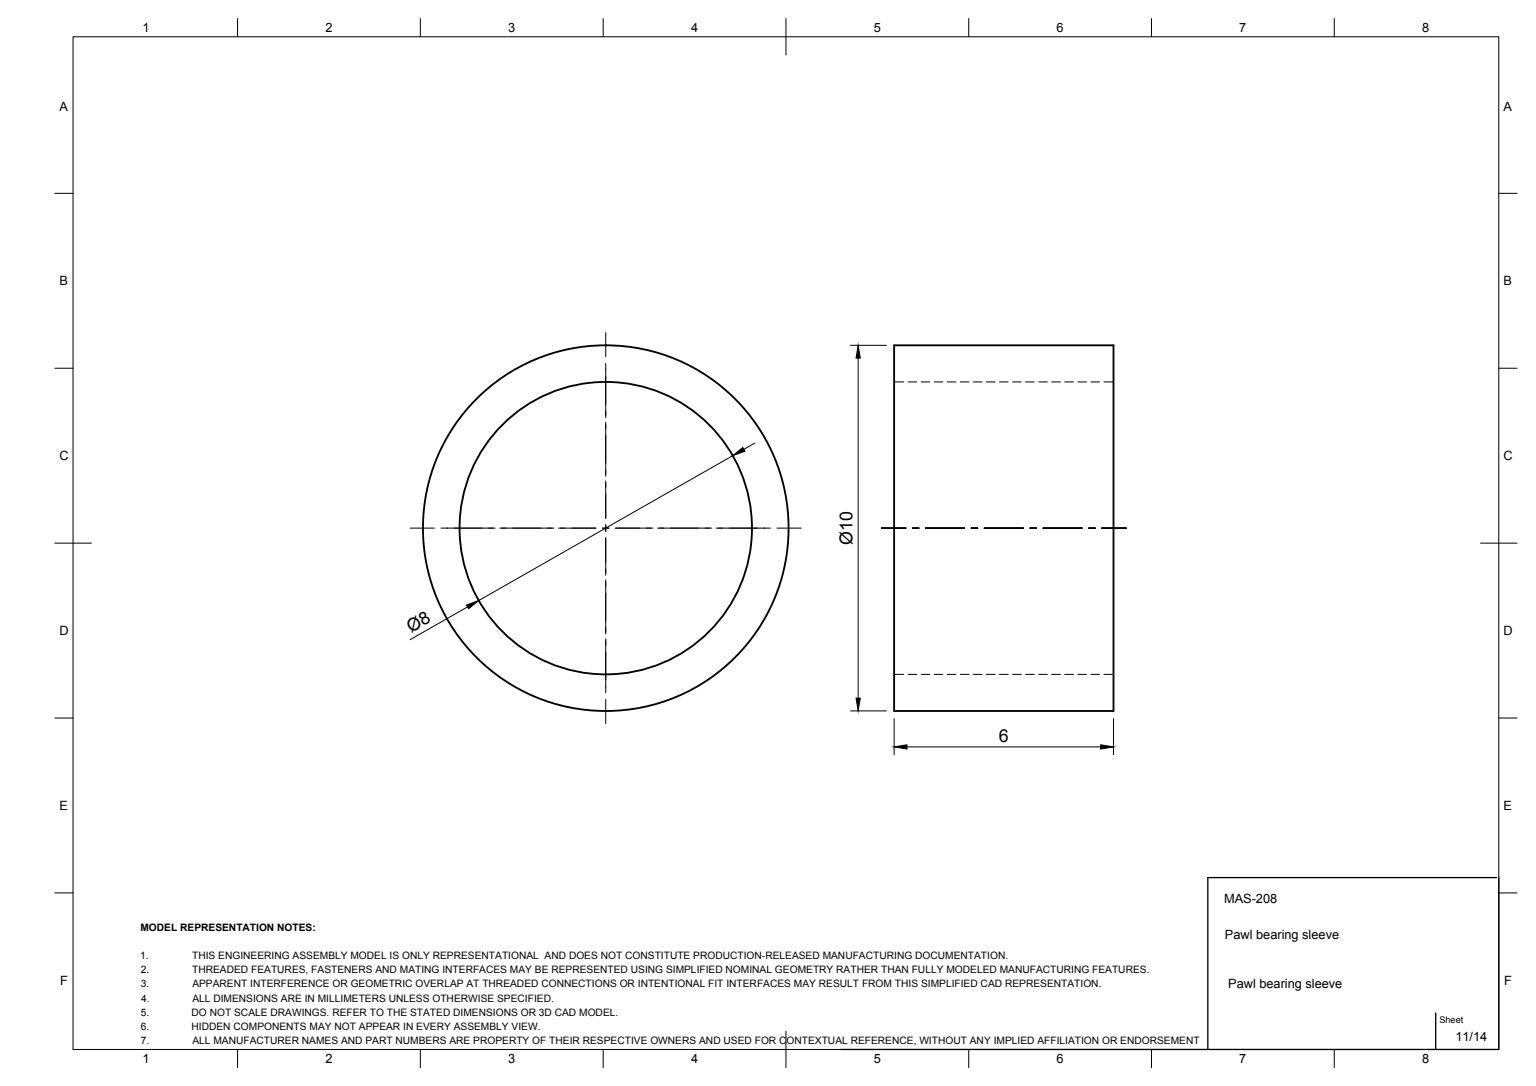
ISO-10303-21;
HEADER;
/* Generated by software containing ST-Developer
 * from STEP Tools, Inc. (www.steptools.com) 
 */

FILE_DESCRIPTION(
/* description */ ('Independent vertical20-tooth ratchet advance with repeated integral-c
ounterweight gravity pawls, swinging drive lever, bronze sleeves and f
ully retained axle stacks.18degpertooth. Native revolutes; geometric c
ycle checking rather than automatic contact/rolling dynamics. Gravity 
closing checked from actual pawl center of mass. Backplate/foot suppor
ts unit. Fits, torque, holding force, wear and life unassigned.'),
/* implementation_level */ '2;1');

FILE_NAME(
/* name */ 'Pawl bearing sleeve.step',
/* time_stamp */ '2026-11-09T06:25:53-08:00',
/* author */ (''),
/* organization */ (''),
/* preprocessor_version */ 'ST-DEVELOPER v20.2',
/* originating_system */ 'Autodesk Translation Framework v15.17.0.0',
/* authorisation */ '');

FILE_SCHEMA (('AUTOMOTIVE_DESIGN { 1 0 10303 214 3 1 1 }'));
ENDSEC;

DATA;
#10=MECHANICAL_DESIGN_GEOMETRIC_PRESENTATION_REPRESENTATION('',(#132),#4643);
#104=SHAPE_REPRESENTATION_RELATIONSHIP('SRR','None',#4709,#118);
#118=ADVANCED_BREP_SHAPE_REPRESENTATION('',(#146),#4638);
#132=STYLED_ITEM('',(#4785),#146);
#146=MANIFOLD_SOLID_BREP('Body1',#2668);
#184=FACE_BOUND('',#616,.T.);
#185=FACE_BOUND('',#618,.T.);
#292=PLANE('',#3026);
#293=PLANE('',#3027);
#431=FACE_OUTER_BOUND('',#613,.T.);
#432=FACE_OUTER_BOUND('',#614,.T.);
#433=FACE_OUTER_BOUND('',#615,.T.);
#434=FACE_OUTER_BOUND('',#617,.T.);
#613=EDGE_LOOP('',(#2401,#2402,#2403,#2404));
#614=EDGE_LOOP('',(#2405,#2406,#2407,#2408));
#615=EDGE_LOOP('',(#2409));
#616=EDGE_LOOP('',(#2410));
#617=EDGE_LOOP('',(#2411));
#618=EDGE_LOOP('',(#2412));
#889=LINE('',#4509,#1151);
#890=LINE('',#4515,#1152);
#1151=VECTOR('',#3721,4.);
#1152=VECTOR('',#3728,5.);
#1221=CIRCLE('',#3021,4.);
#1222=CIRCLE('',#3022,4.);
#1223=CIRCLE('',#3024,5.);
#1224=CIRCLE('',#3025,5.);
#1441=VERTEX_POINT('',#4506);
#1442=VERTEX_POINT('',#4508);
#1443=VERTEX_POINT('',#4512);
#1444=VERTEX_POINT('',#4514);
#1765=EDGE_CURVE('',#1441,#1441,#1221,.T.);
#1766=EDGE_CURVE('',#1441,#1442,#889,.T.);
#1767=EDGE_CURVE('',#1442,#1442,#1222,.T.);
#1768=EDGE_CURVE('',#1443,#1443,#1223,.T.);
#1769=EDGE_CURVE('',#1443,#1444,#890,.T.);
#1770=EDGE_CURVE('',#1444,#1444,#1224,.T.);
#2401=ORIENTED_EDGE('',*,*,#1765,.F.);
#2402=ORIENTED_EDGE('',*,*,#1766,.T.);
#2403=ORIENTED_EDGE('',*,*,#1767,.T.);
#2404=ORIENTED_EDGE('',*,*,#1766,.F.);
#2405=ORIENTED_EDGE('',*,*,#1768,.F.);
#2406=ORIENTED_EDGE('',*,*,#1769,.T.);
#2407=ORIENTED_EDGE('',*,*,#1770,.T.);
#2408=ORIENTED_EDGE('',*,*,#1769,.F.);
#2409=ORIENTED_EDGE('',*,*,#1768,.T.);
#2410=ORIENTED_EDGE('',*,*,#1765,.T.);
#2411=ORIENTED_EDGE('',*,*,#1770,.F.);
#2412=ORIENTED_EDGE('',*,*,#1767,.F.);
#2500=CYLINDRICAL_SURFACE('',#3020,4.);
#2501=CYLINDRICAL_SURFACE('',#3023,5.);
#2637=ADVANCED_FACE('',(#431),#2500,.F.);
#2638=ADVANCED_FACE('',(#432),#2501,.T.);
#2639=ADVANCED_FACE('',(#433,#184),#292,.T.);
#2640=ADVANCED_FACE('',(#434,#185),#293,.F.);
#2668=CLOSED_SHELL('',(#2637,#2638,#2639,#2640));
#3019=AXIS2_PLACEMENT_3D('',#4504,#3715,#3716);
#3020=AXIS2_PLACEMENT_3D('',#4505,#3717,#3718);
#3021=AXIS2_PLACEMENT_3D('',#4507,#3719,#3720);
#3022=AXIS2_PLACEMENT_3D('',#4510,#3722,#3723);
#3023=AXIS2_PLACEMENT_3D('',#4511,#3724,#3725);
#3024=AXIS2_PLACEMENT_3D('',#4513,#3726,#3727);
#3025=AXIS2_PLACEMENT_3D('',#4516,#3729,#3730);
#3026=AXIS2_PLACEMENT_3D('',#4517,#3731,#3732);
#3027=AXIS2_PLACEMENT_3D('',#4518,#3733,#3734);
#3715=DIRECTION('axis',(0.,0.,1.));
#3716=DIRECTION('refdir',(1.,0.,0.));
#3717=DIRECTION('center_axis',(0.,0.,1.));
#3718=DIRECTION('ref_axis',(1.,0.,0.));
#3719=DIRECTION('center_axis',(0.,0.,-1.));
#3720=DIRECTION('ref_axis',(1.,0.,0.));
#3721=DIRECTION('',(0.,0.,-1.));
#3722=DIRECTION('center_axis',(0.,0.,-1.));
#3723=DIRECTION('ref_axis',(1.,0.,0.));
#3724=DIRECTION('center_axis',(0.,0.,1.));
#3725=DIRECTION('ref_axis',(1.,0.,0.));
#3726=DIRECTION('center_axis',(0.,0.,1.));
#3727=DIRECTION('ref_axis',(1.,0.,0.));
#3728=DIRECTION('',(0.,0.,-1.));
#3729=DIRECTION('center_axis',(0.,0.,1.));
#3730=DIRECTION('ref_axis',(1.,0.,0.));
#3731=DIRECTION('center_axis',(0.,0.,1.));
#3732=DIRECTION('ref_axis',(1.,0.,0.));
#3733=DIRECTION('center_axis',(0.,0.,1.));
#3734=DIRECTION('ref_axis',(1.,0.,0.));
#4504=CARTESIAN_POINT('',(0.,0.,0.));
#4505=CARTESIAN_POINT('Origin',(0.,0.,0.));
#4506=CARTESIAN_POINT('',(-4.,-4.89858719658941E-16,6.));
#4507=CARTESIAN_POINT('Origin',(0.,0.,6.));
#4508=CARTESIAN_POINT('',(-4.,-4.89858719658941E-16,0.));
#4509=CARTESIAN_POINT('',(-4.,-4.89858719658941E-16,0.));
#4510=CARTESIAN_POINT('Origin',(0.,0.,0.));
#4511=CARTESIAN_POINT('Origin',(0.,0.,0.));
#4512=CARTESIAN_POINT('',(-5.,-6.12323399573677E-16,6.));
#4513=CARTESIAN_POINT('Origin',(0.,0.,6.));
#4514=CARTESIAN_POINT('',(-5.,-6.12323399573677E-16,0.));
#4515=CARTESIAN_POINT('',(-5.,-6.12323399573677E-16,0.));
#4516=CARTESIAN_POINT('Origin',(0.,0.,0.));
#4517=CARTESIAN_POINT('Origin',(0.,0.,6.));
#4518=CARTESIAN_POINT('Origin',(0.,0.,0.));
#4622=UNCERTAINTY_MEASURE_WITH_UNIT(LENGTH_MEASURE(0.01),#4644,
'DISTANCE_ACCURACY_VALUE',
'Maximum model space distance between geometric entities at asserted c
onnectivities');
#4627=UNCERTAINTY_MEASURE_WITH_UNIT(LENGTH_MEASURE(0.01),#4644,
'DISTANCE_ACCURACY_VALUE',
'Maximum model space distance between geometric entities at asserted c
onnectivities');
#4638=(
GEOMETRIC_REPRESENTATION_CONTEXT(3)
GLOBAL_UNCERTAINTY_ASSIGNED_CONTEXT((#4622))
GLOBAL_UNIT_ASSIGNED_CONTEXT((#4644,#4646,#4647))
REPRESENTATION_CONTEXT('','3D')
);
#4643=(
GEOMETRIC_REPRESENTATION_CONTEXT(3)
GLOBAL_UNCERTAINTY_ASSIGNED_CONTEXT((#4627))
GLOBAL_UNIT_ASSIGNED_CONTEXT((#4644,#4646,#4647))
REPRESENTATION_CONTEXT('','3D')
);
#4644=(
LENGTH_UNIT()
NAMED_UNIT(*)
SI_UNIT(.MILLI.,.METRE.)
);
#4646=(
NAMED_UNIT(*)
PLANE_ANGLE_UNIT()
SI_UNIT($,.RADIAN.)
);
#4647=(
NAMED_UNIT(*)
SI_UNIT($,.STERADIAN.)
SOLID_ANGLE_UNIT()
);
#4658=SHAPE_DEFINITION_REPRESENTATION(#4673,#4709);
#4673=PRODUCT_DEFINITION_SHAPE('',$,#4725);
#4709=SHAPE_REPRESENTATION('',(#3019),#4638);
#4714=PRODUCT_DEFINITION_CONTEXT('part definition',#4761,'design');
#4725=PRODUCT_DEFINITION('Pawl bearing sleeve','Pawl bearing sleeve',#4740,
#4714);
#4740=PRODUCT_DEFINITION_FORMATION('',$,#4773);
#4761=APPLICATION_CONTEXT(
'Core Data for Automotive Mechanical Design Process');
#4762=PRODUCT_CONTEXT('part definition',#4761,'mechanical');
#4773=PRODUCT('Pawl bearing sleeve','Pawl bearing sleeve',$,(#4762));
#4785=PRESENTATION_STYLE_ASSIGNMENT((#4794));
#4794=SURFACE_STYLE_USAGE(.BOTH.,#4803);
#4803=SURFACE_SIDE_STYLE('',(#4812));
#4812=SURFACE_STYLE_FILL_AREA(#4821);
#4821=FILL_AREA_STYLE('Bearing light gray',(#4830));
#4830=FILL_AREA_STYLE_COLOUR('Bearing light gray',#4839);
#4839=COLOUR_RGB('Bearing light gray',0.725490196078431,0.752941176470588,
0.792156862745098);
ENDSEC;
END-ISO-10303-21;
